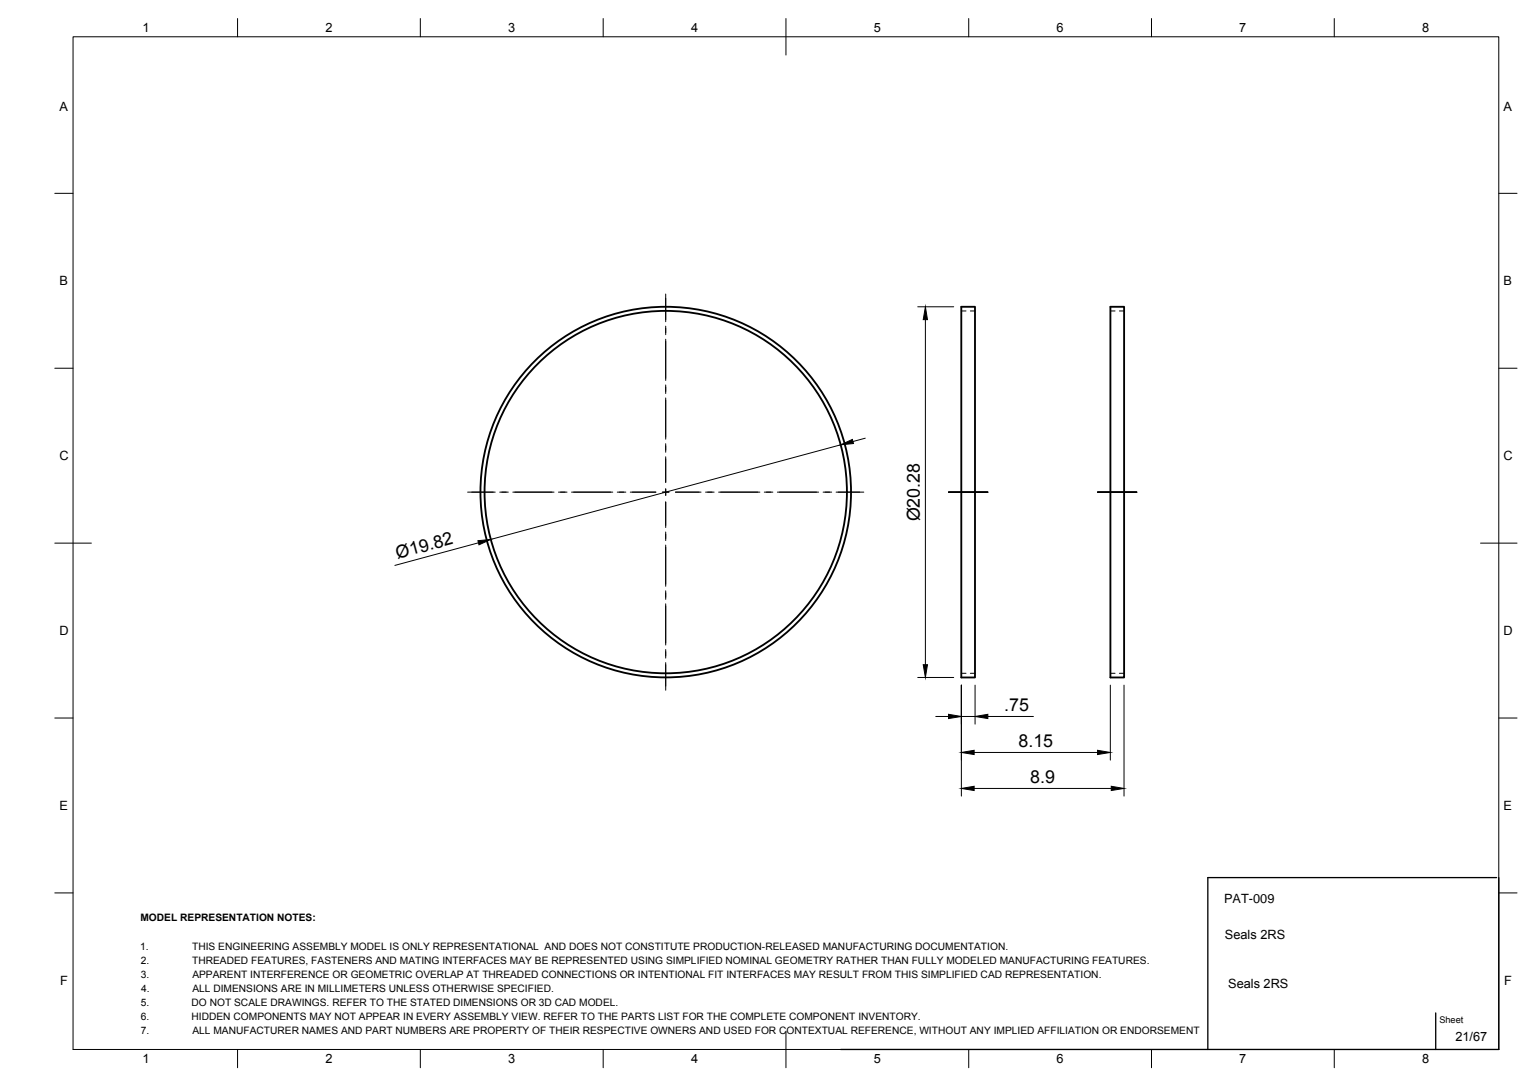
ISO-10303-21;
HEADER;
/* Generated by software containing ST-Developer
 * from STEP Tools, Inc. (www.steptools.com) 
 */

FILE_DESCRIPTION(
/* description */ ('Bell-crank linkage with push rods'),
/* implementation_level */ '2;1');

FILE_NAME(
/* name */ 'Seals 2RS.step',
/* time_stamp */ '2026-10-28T03:25:15-07:00',
/* author */ (''),
/* organization */ (''),
/* preprocessor_version */ 'ST-DEVELOPER v20.2',
/* originating_system */ 'Autodesk Translation Framework v15.17.0.0',
/* authorisation */ '');

FILE_SCHEMA (('AUTOMOTIVE_DESIGN { 1 0 10303 214 3 1 1 }'));
ENDSEC;

DATA;
#10=MECHANICAL_DESIGN_GEOMETRIC_PRESENTATION_REPRESENTATION('',(#625,#626),#16678);
#510=SHAPE_REPRESENTATION_RELATIONSHIP('SRR','None',#16927,#564);
#564=ADVANCED_BREP_SHAPE_REPRESENTATION('',(#686,#687),#16632);
#625=STYLED_ITEM('',(#17291),#686);
#626=STYLED_ITEM('',(#17291),#687);
#686=MANIFOLD_SOLID_BREP('Body1',#8816);
#687=MANIFOLD_SOLID_BREP('Body2',#8817);
#818=FACE_BOUND('',#2069,.T.);
#819=FACE_BOUND('',#2072,.T.);
#820=FACE_BOUND('',#2075,.T.);
#821=FACE_BOUND('',#2078,.T.);
#1067=PLANE('',#9901);
#1068=PLANE('',#9906);
#1069=PLANE('',#9909);
#1070=PLANE('',#9914);
#1453=FACE_OUTER_BOUND('',#2068,.T.);
#1454=FACE_OUTER_BOUND('',#2070,.T.);
#1455=FACE_OUTER_BOUND('',#2071,.T.);
#1456=FACE_OUTER_BOUND('',#2073,.T.);
#1457=FACE_OUTER_BOUND('',#2074,.T.);
#1458=FACE_OUTER_BOUND('',#2076,.T.);
#1459=FACE_OUTER_BOUND('',#2077,.T.);
#1460=FACE_OUTER_BOUND('',#2079,.T.);
#2068=EDGE_LOOP('',(#6863));
#2069=EDGE_LOOP('',(#6864));
#2070=EDGE_LOOP('',(#6865,#6866,#6867,#6868));
#2071=EDGE_LOOP('',(#6869));
#2072=EDGE_LOOP('',(#6870));
#2073=EDGE_LOOP('',(#6871,#6872,#6873,#6874));
#2074=EDGE_LOOP('',(#6875));
#2075=EDGE_LOOP('',(#6876));
#2076=EDGE_LOOP('',(#6877,#6878,#6879,#6880));
#2077=EDGE_LOOP('',(#6881));
#2078=EDGE_LOOP('',(#6882));
#2079=EDGE_LOOP('',(#6883,#6884,#6885,#6886));
#2751=LINE('',#15036,#3300);
#2752=LINE('',#15041,#3301);
#2753=LINE('',#15050,#3302);
#2754=LINE('',#15055,#3303);
#3300=VECTOR('',#11753,1.013815);
#3301=VECTOR('',#11760,0.991185);
#3302=VECTOR('',#11771,1.013815);
#3303=VECTOR('',#11778,0.991185);
#3853=CIRCLE('',#9902,1.013815);
#3854=CIRCLE('',#9903,0.991185);
#3855=CIRCLE('',#9905,1.013815);
#3856=CIRCLE('',#9907,0.991185);
#3857=CIRCLE('',#9910,1.013815);
#3858=CIRCLE('',#9911,0.991185);
#3859=CIRCLE('',#9913,1.013815);
#3860=CIRCLE('',#9915,0.991185);
#4435=VERTEX_POINT('',#15029);
#4436=VERTEX_POINT('',#15031);
#4437=VERTEX_POINT('',#15034);
#4438=VERTEX_POINT('',#15038);
#4439=VERTEX_POINT('',#15043);
#4440=VERTEX_POINT('',#15045);
#4441=VERTEX_POINT('',#15048);
#4442=VERTEX_POINT('',#15052);
#5309=EDGE_CURVE('',#4435,#4435,#3853,.T.);
#5310=EDGE_CURVE('',#4436,#4436,#3854,.T.);
#5311=EDGE_CURVE('',#4437,#4437,#3855,.T.);
#5312=EDGE_CURVE('',#4437,#4435,#2751,.T.);
#5313=EDGE_CURVE('',#4438,#4438,#3856,.T.);
#5314=EDGE_CURVE('',#4438,#4436,#2752,.T.);
#5315=EDGE_CURVE('',#4439,#4439,#3857,.T.);
#5316=EDGE_CURVE('',#4440,#4440,#3858,.T.);
#5317=EDGE_CURVE('',#4441,#4441,#3859,.T.);
#5318=EDGE_CURVE('',#4441,#4439,#2753,.T.);
#5319=EDGE_CURVE('',#4442,#4442,#3860,.T.);
#5320=EDGE_CURVE('',#4442,#4440,#2754,.T.);
#6863=ORIENTED_EDGE('',*,*,#5309,.F.);
#6864=ORIENTED_EDGE('',*,*,#5310,.T.);
#6865=ORIENTED_EDGE('',*,*,#5311,.F.);
#6866=ORIENTED_EDGE('',*,*,#5312,.T.);
#6867=ORIENTED_EDGE('',*,*,#5309,.T.);
#6868=ORIENTED_EDGE('',*,*,#5312,.F.);
#6869=ORIENTED_EDGE('',*,*,#5311,.T.);
#6870=ORIENTED_EDGE('',*,*,#5313,.F.);
#6871=ORIENTED_EDGE('',*,*,#5313,.T.);
#6872=ORIENTED_EDGE('',*,*,#5314,.T.);
#6873=ORIENTED_EDGE('',*,*,#5310,.F.);
#6874=ORIENTED_EDGE('',*,*,#5314,.F.);
#6875=ORIENTED_EDGE('',*,*,#5315,.F.);
#6876=ORIENTED_EDGE('',*,*,#5316,.T.);
#6877=ORIENTED_EDGE('',*,*,#5317,.F.);
#6878=ORIENTED_EDGE('',*,*,#5318,.T.);
#6879=ORIENTED_EDGE('',*,*,#5315,.T.);
#6880=ORIENTED_EDGE('',*,*,#5318,.F.);
#6881=ORIENTED_EDGE('',*,*,#5317,.T.);
#6882=ORIENTED_EDGE('',*,*,#5319,.F.);
#6883=ORIENTED_EDGE('',*,*,#5319,.T.);
#6884=ORIENTED_EDGE('',*,*,#5320,.T.);
#6885=ORIENTED_EDGE('',*,*,#5316,.F.);
#6886=ORIENTED_EDGE('',*,*,#5320,.F.);
#8147=CYLINDRICAL_SURFACE('',#9904,1.013815);
#8148=CYLINDRICAL_SURFACE('',#9908,0.991185);
#8149=CYLINDRICAL_SURFACE('',#9912,1.013815);
#8150=CYLINDRICAL_SURFACE('',#9916,0.991185);
#8478=ADVANCED_FACE('',(#1453,#818),#1067,.T.);
#8479=ADVANCED_FACE('',(#1454),#8147,.T.);
#8480=ADVANCED_FACE('',(#1455,#819),#1068,.T.);
#8481=ADVANCED_FACE('',(#1456),#8148,.F.);
#8482=ADVANCED_FACE('',(#1457,#820),#1069,.T.);
#8483=ADVANCED_FACE('',(#1458),#8149,.T.);
#8484=ADVANCED_FACE('',(#1459,#821),#1070,.T.);
#8485=ADVANCED_FACE('',(#1460),#8150,.F.);
#8816=CLOSED_SHELL('',(#8478,#8479,#8480,#8481));
#8817=CLOSED_SHELL('',(#8482,#8483,#8484,#8485));
#9900=AXIS2_PLACEMENT_3D('',#15027,#11741,#11742);
#9901=AXIS2_PLACEMENT_3D('',#15028,#11743,#11744);
#9902=AXIS2_PLACEMENT_3D('',#15030,#11745,#11746);
#9903=AXIS2_PLACEMENT_3D('',#15032,#11747,#11748);
#9904=AXIS2_PLACEMENT_3D('',#15033,#11749,#11750);
#9905=AXIS2_PLACEMENT_3D('',#15035,#11751,#11752);
#9906=AXIS2_PLACEMENT_3D('',#15037,#11754,#11755);
#9907=AXIS2_PLACEMENT_3D('',#15039,#11756,#11757);
#9908=AXIS2_PLACEMENT_3D('',#15040,#11758,#11759);
#9909=AXIS2_PLACEMENT_3D('',#15042,#11761,#11762);
#9910=AXIS2_PLACEMENT_3D('',#15044,#11763,#11764);
#9911=AXIS2_PLACEMENT_3D('',#15046,#11765,#11766);
#9912=AXIS2_PLACEMENT_3D('',#15047,#11767,#11768);
#9913=AXIS2_PLACEMENT_3D('',#15049,#11769,#11770);
#9914=AXIS2_PLACEMENT_3D('',#15051,#11772,#11773);
#9915=AXIS2_PLACEMENT_3D('',#15053,#11774,#11775);
#9916=AXIS2_PLACEMENT_3D('',#15054,#11776,#11777);
#11741=DIRECTION('axis',(0.,0.,1.));
#11742=DIRECTION('refdir',(1.,0.,0.));
#11743=DIRECTION('center_axis',(0.,1.,0.));
#11744=DIRECTION('ref_axis',(0.,0.,1.));
#11745=DIRECTION('center_axis',(0.,-1.,0.));
#11746=DIRECTION('ref_axis',(1.,0.,0.));
#11747=DIRECTION('center_axis',(0.,-1.,0.));
#11748=DIRECTION('ref_axis',(1.,0.,0.));
#11749=DIRECTION('center_axis',(0.,-1.,0.));
#11750=DIRECTION('ref_axis',(1.,0.,0.));
#11751=DIRECTION('center_axis',(0.,-1.,0.));
#11752=DIRECTION('ref_axis',(1.,0.,0.));
#11753=DIRECTION('',(0.,1.,0.));
#11754=DIRECTION('center_axis',(0.,-1.,0.));
#11755=DIRECTION('ref_axis',(0.,0.,-1.));
#11756=DIRECTION('center_axis',(0.,-1.,0.));
#11757=DIRECTION('ref_axis',(1.,0.,0.));
#11758=DIRECTION('center_axis',(0.,-1.,0.));
#11759=DIRECTION('ref_axis',(1.,0.,0.));
#11760=DIRECTION('',(0.,1.,0.));
#11761=DIRECTION('center_axis',(0.,1.,0.));
#11762=DIRECTION('ref_axis',(0.,0.,1.));
#11763=DIRECTION('center_axis',(0.,-1.,0.));
#11764=DIRECTION('ref_axis',(1.,0.,0.));
#11765=DIRECTION('center_axis',(0.,-1.,0.));
#11766=DIRECTION('ref_axis',(1.,0.,0.));
#11767=DIRECTION('center_axis',(0.,-1.,0.));
#11768=DIRECTION('ref_axis',(1.,0.,0.));
#11769=DIRECTION('center_axis',(0.,-1.,0.));
#11770=DIRECTION('ref_axis',(1.,0.,0.));
#11771=DIRECTION('',(0.,1.,0.));
#11772=DIRECTION('center_axis',(0.,-1.,0.));
#11773=DIRECTION('ref_axis',(0.,0.,-1.));
#11774=DIRECTION('center_axis',(0.,-1.,0.));
#11775=DIRECTION('ref_axis',(1.,0.,0.));
#11776=DIRECTION('center_axis',(0.,-1.,0.));
#11777=DIRECTION('ref_axis',(1.,0.,0.));
#11778=DIRECTION('',(0.,1.,0.));
#15027=CARTESIAN_POINT('',(0.,0.,0.));
#15028=CARTESIAN_POINT('Origin',(1.013815,0.445,0.));
#15029=CARTESIAN_POINT('',(-1.013815,0.445,-1.24156529467757E-16));
#15030=CARTESIAN_POINT('Origin',(0.,0.445,0.));
#15031=CARTESIAN_POINT('',(-0.991185,0.445,-1.21385153761287E-16));
#15032=CARTESIAN_POINT('Origin',(0.,0.445,0.));
#15033=CARTESIAN_POINT('Origin',(0.,0.4075,0.));
#15034=CARTESIAN_POINT('',(-1.013815,0.37,-1.24156529467757E-16));
#15035=CARTESIAN_POINT('Origin',(0.,0.37,0.));
#15036=CARTESIAN_POINT('',(-1.013815,0.4075,-1.24156529467757E-16));
#15037=CARTESIAN_POINT('Origin',(0.991185,0.37,0.));
#15038=CARTESIAN_POINT('',(-0.991185,0.37,-1.21385153761287E-16));
#15039=CARTESIAN_POINT('Origin',(0.,0.37,0.));
#15040=CARTESIAN_POINT('Origin',(0.,0.4075,0.));
#15041=CARTESIAN_POINT('',(-0.991185,0.4075,-1.21385153761287E-16));
#15042=CARTESIAN_POINT('Origin',(1.013815,-0.37,0.));
#15043=CARTESIAN_POINT('',(-1.013815,-0.37,-1.24156529467757E-16));
#15044=CARTESIAN_POINT('Origin',(0.,-0.37,0.));
#15045=CARTESIAN_POINT('',(-0.991185,-0.37,-1.21385153761287E-16));
#15046=CARTESIAN_POINT('Origin',(0.,-0.37,0.));
#15047=CARTESIAN_POINT('Origin',(0.,-0.4075,0.));
#15048=CARTESIAN_POINT('',(-1.013815,-0.445,-1.24156529467757E-16));
#15049=CARTESIAN_POINT('Origin',(0.,-0.445,0.));
#15050=CARTESIAN_POINT('',(-1.013815,-0.4075,-1.24156529467757E-16));
#15051=CARTESIAN_POINT('Origin',(0.991185,-0.445,0.));
#15052=CARTESIAN_POINT('',(-0.991185,-0.445,-1.21385153761287E-16));
#15053=CARTESIAN_POINT('Origin',(0.,-0.445,0.));
#15054=CARTESIAN_POINT('Origin',(0.,-0.4075,0.));
#15055=CARTESIAN_POINT('',(-0.991185,-0.4075,-1.21385153761287E-16));
#16568=UNCERTAINTY_MEASURE_WITH_UNIT(LENGTH_MEASURE(0.001),#16679,
'DISTANCE_ACCURACY_VALUE',
'Maximum model space distance between geometric entities at asserted c
onnectivities');
#16614=UNCERTAINTY_MEASURE_WITH_UNIT(LENGTH_MEASURE(0.001),#16679,
'DISTANCE_ACCURACY_VALUE',
'Maximum model space distance between geometric entities at asserted c
onnectivities');
#16632=(
GEOMETRIC_REPRESENTATION_CONTEXT(3)
GLOBAL_UNCERTAINTY_ASSIGNED_CONTEXT((#16568))
GLOBAL_UNIT_ASSIGNED_CONTEXT((#16679,#16681,#16682))
REPRESENTATION_CONTEXT('','3D')
);
#16678=(
GEOMETRIC_REPRESENTATION_CONTEXT(3)
GLOBAL_UNCERTAINTY_ASSIGNED_CONTEXT((#16614))
GLOBAL_UNIT_ASSIGNED_CONTEXT((#16679,#16681,#16682))
REPRESENTATION_CONTEXT('','3D')
);
#16679=(
LENGTH_UNIT()
NAMED_UNIT(*)
SI_UNIT(.CENTI.,.METRE.)
);
#16681=(
NAMED_UNIT(*)
PLANE_ANGLE_UNIT()
SI_UNIT($,.RADIAN.)
);
#16682=(
NAMED_UNIT(*)
SI_UNIT($,.STERADIAN.)
SOLID_ANGLE_UNIT()
);
#16700=SHAPE_DEFINITION_REPRESENTATION(#16763,#16927);
#16763=PRODUCT_DEFINITION_SHAPE('',$,#16991);
#16927=SHAPE_REPRESENTATION('',(#9900),#16632);
#16973=PRODUCT_DEFINITION_CONTEXT('part definition',#17164,'design');
#16991=PRODUCT_DEFINITION('Seals 2RS','Seals 2RS',#17054,#16973);
#17054=PRODUCT_DEFINITION_FORMATION('',$,#17183);
#17164=APPLICATION_CONTEXT(
'Core Data for Automotive Mechanical Design Process');
#17165=PRODUCT_CONTEXT('part definition',#17164,'mechanical');
#17183=PRODUCT('Seals 2RS','Seals 2RS','Seals 2RS',(#17165));
#17285=COLOUR_RGB('Grey',0.48,0.52,0.57);
#17286=FILL_AREA_STYLE_COLOUR('',#17285);
#17287=FILL_AREA_STYLE('',(#17286));
#17288=SURFACE_STYLE_FILL_AREA(#17287);
#17289=SURFACE_SIDE_STYLE('',(#17288));
#17290=SURFACE_STYLE_USAGE(.BOTH.,#17289);
#17291=PRESENTATION_STYLE_ASSIGNMENT((#17290));
ENDSEC;
END-ISO-10303-21;
